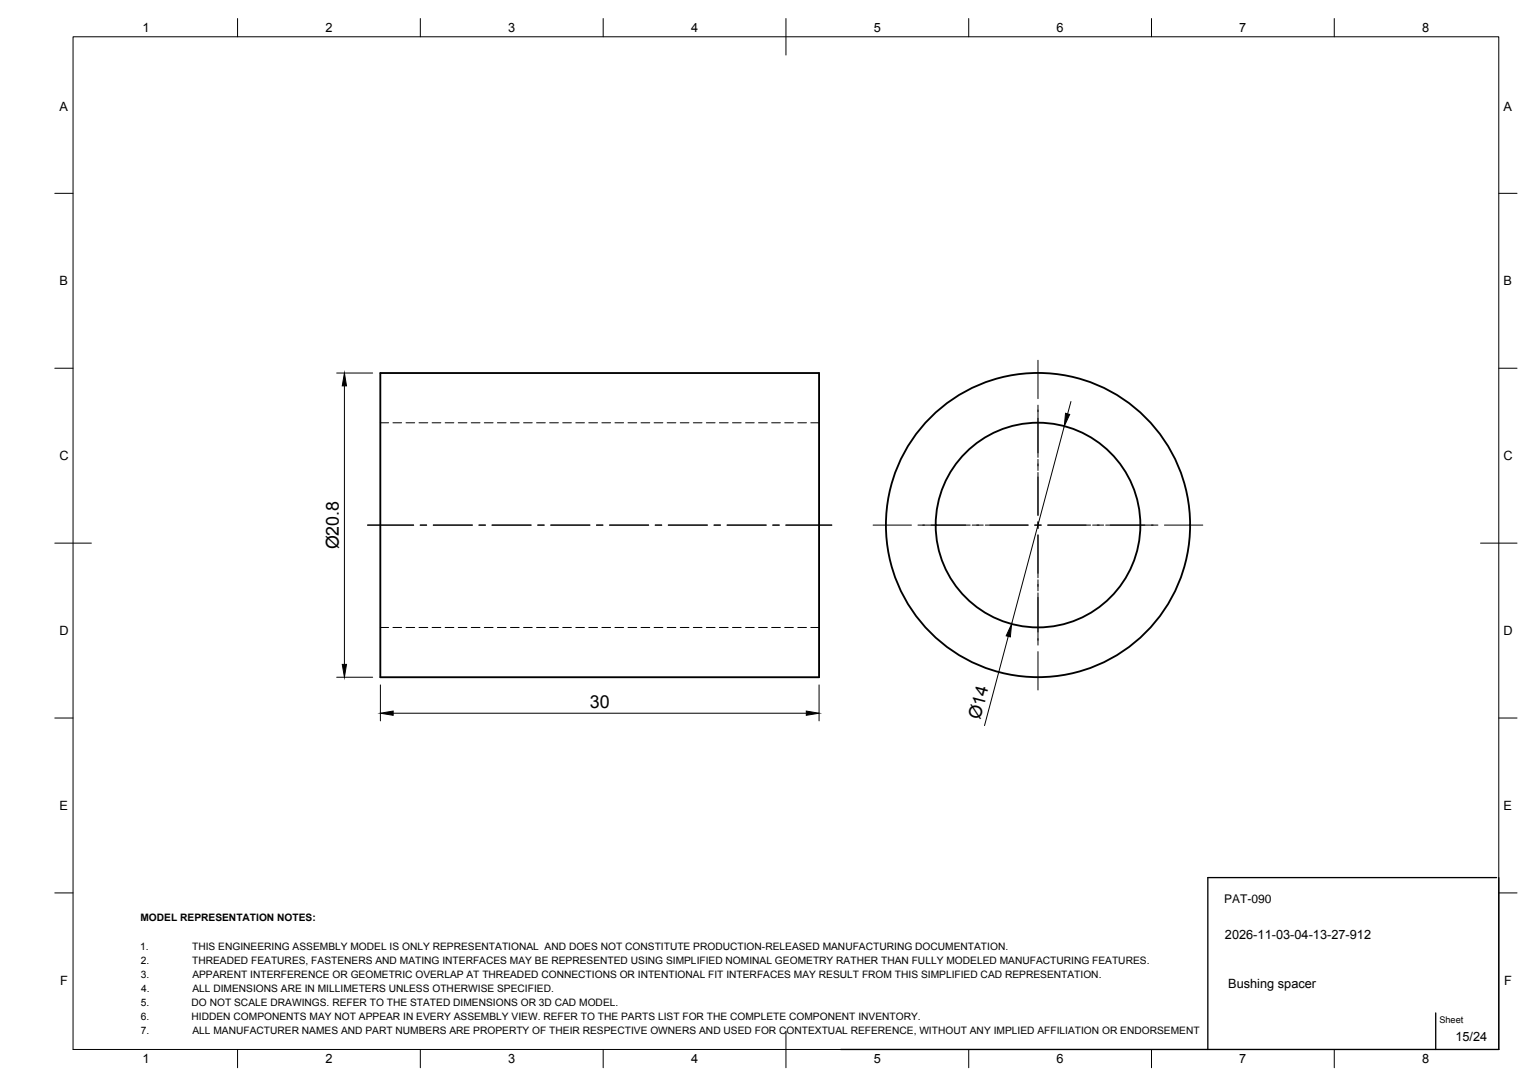
ISO-10303-21;
HEADER;
/* Generated by software containing ST-Developer
 * from STEP Tools, Inc. (www.steptools.com) 
 */

FILE_DESCRIPTION(
/* description */ ('Round-Shaft Linear Stage with Ball Bushings'),
/* implementation_level */ '2;1');

FILE_NAME(
/* name */ 'Bushing spacer.step',
/* time_stamp */ '2026-10-27T10:47:55-07:00',
/* author */ (''),
/* organization */ (''),
/* preprocessor_version */ 'ST-DEVELOPER v20.2',
/* originating_system */ 'Autodesk Translation Framework v15.17.0.0',
/* authorisation */ '');

FILE_SCHEMA (('AUTOMOTIVE_DESIGN { 1 0 10303 214 3 1 1 }'));
ENDSEC;

DATA;
#10=MECHANICAL_DESIGN_GEOMETRIC_PRESENTATION_REPRESENTATION('',(#311),#7835);
#269=SHAPE_REPRESENTATION_RELATIONSHIP('SRR','None',#7958,#290);
#290=ADVANCED_BREP_SHAPE_REPRESENTATION('',(#331),#7822);
#311=STYLED_ITEM('',(#8158),#331);
#331=MANIFOLD_SOLID_BREP('Body1',#4402);
#403=FACE_BOUND('',#1069,.T.);
#404=FACE_BOUND('',#1071,.T.);
#540=PLANE('',#4891);
#541=PLANE('',#4892);
#746=FACE_OUTER_BOUND('',#1066,.T.);
#747=FACE_OUTER_BOUND('',#1067,.T.);
#748=FACE_OUTER_BOUND('',#1068,.T.);
#749=FACE_OUTER_BOUND('',#1070,.T.);
#1066=EDGE_LOOP('',(#3542,#3543,#3544,#3545));
#1067=EDGE_LOOP('',(#3546,#3547,#3548,#3549));
#1068=EDGE_LOOP('',(#3550));
#1069=EDGE_LOOP('',(#3551));
#1070=EDGE_LOOP('',(#3552));
#1071=EDGE_LOOP('',(#3553));
#1430=LINE('',#7172,#1770);
#1431=LINE('',#7178,#1771);
#1770=VECTOR('',#5833,0.7);
#1771=VECTOR('',#5840,1.04);
#2022=CIRCLE('',#4886,0.7);
#2023=CIRCLE('',#4887,0.7);
#2024=CIRCLE('',#4889,1.04);
#2025=CIRCLE('',#4890,1.04);
#2299=VERTEX_POINT('',#7169);
#2300=VERTEX_POINT('',#7171);
#2301=VERTEX_POINT('',#7175);
#2302=VERTEX_POINT('',#7177);
#2739=EDGE_CURVE('',#2299,#2299,#2022,.T.);
#2740=EDGE_CURVE('',#2299,#2300,#1430,.T.);
#2741=EDGE_CURVE('',#2300,#2300,#2023,.T.);
#2742=EDGE_CURVE('',#2301,#2301,#2024,.T.);
#2743=EDGE_CURVE('',#2301,#2302,#1431,.T.);
#2744=EDGE_CURVE('',#2302,#2302,#2025,.T.);
#3542=ORIENTED_EDGE('',*,*,#2739,.F.);
#3543=ORIENTED_EDGE('',*,*,#2740,.T.);
#3544=ORIENTED_EDGE('',*,*,#2741,.T.);
#3545=ORIENTED_EDGE('',*,*,#2740,.F.);
#3546=ORIENTED_EDGE('',*,*,#2742,.F.);
#3547=ORIENTED_EDGE('',*,*,#2743,.T.);
#3548=ORIENTED_EDGE('',*,*,#2744,.T.);
#3549=ORIENTED_EDGE('',*,*,#2743,.F.);
#3550=ORIENTED_EDGE('',*,*,#2742,.T.);
#3551=ORIENTED_EDGE('',*,*,#2739,.T.);
#3552=ORIENTED_EDGE('',*,*,#2744,.F.);
#3553=ORIENTED_EDGE('',*,*,#2741,.F.);
#4096=CYLINDRICAL_SURFACE('',#4885,0.7);
#4097=CYLINDRICAL_SURFACE('',#4888,1.04);
#4265=ADVANCED_FACE('',(#746),#4096,.F.);
#4266=ADVANCED_FACE('',(#747),#4097,.T.);
#4267=ADVANCED_FACE('',(#748,#403),#540,.T.);
#4268=ADVANCED_FACE('',(#749,#404),#541,.F.);
#4402=CLOSED_SHELL('',(#4265,#4266,#4267,#4268));
#4884=AXIS2_PLACEMENT_3D('',#7167,#5827,#5828);
#4885=AXIS2_PLACEMENT_3D('',#7168,#5829,#5830);
#4886=AXIS2_PLACEMENT_3D('',#7170,#5831,#5832);
#4887=AXIS2_PLACEMENT_3D('',#7173,#5834,#5835);
#4888=AXIS2_PLACEMENT_3D('',#7174,#5836,#5837);
#4889=AXIS2_PLACEMENT_3D('',#7176,#5838,#5839);
#4890=AXIS2_PLACEMENT_3D('',#7179,#5841,#5842);
#4891=AXIS2_PLACEMENT_3D('',#7180,#5843,#5844);
#4892=AXIS2_PLACEMENT_3D('',#7181,#5845,#5846);
#5827=DIRECTION('axis',(0.,0.,1.));
#5828=DIRECTION('refdir',(1.,0.,0.));
#5829=DIRECTION('center_axis',(1.,0.,0.));
#5830=DIRECTION('ref_axis',(0.,0.,-1.));
#5831=DIRECTION('center_axis',(-1.,0.,0.));
#5832=DIRECTION('ref_axis',(0.,0.,-1.));
#5833=DIRECTION('',(-1.,0.,0.));
#5834=DIRECTION('center_axis',(-1.,0.,0.));
#5835=DIRECTION('ref_axis',(0.,0.,-1.));
#5836=DIRECTION('center_axis',(1.,0.,0.));
#5837=DIRECTION('ref_axis',(0.,0.,-1.));
#5838=DIRECTION('center_axis',(1.,0.,0.));
#5839=DIRECTION('ref_axis',(0.,0.,-1.));
#5840=DIRECTION('',(-1.,0.,0.));
#5841=DIRECTION('center_axis',(1.,0.,0.));
#5842=DIRECTION('ref_axis',(0.,0.,-1.));
#5843=DIRECTION('center_axis',(1.,0.,0.));
#5844=DIRECTION('ref_axis',(0.,0.,-1.));
#5845=DIRECTION('center_axis',(1.,0.,0.));
#5846=DIRECTION('ref_axis',(0.,0.,-1.));
#7167=CARTESIAN_POINT('',(0.,0.,0.));
#7168=CARTESIAN_POINT('Origin',(13.5,-4.,3.3));
#7169=CARTESIAN_POINT('',(16.5,-4.,4.));
#7170=CARTESIAN_POINT('Origin',(16.5,-4.,3.3));
#7171=CARTESIAN_POINT('',(13.5,-4.,4.));
#7172=CARTESIAN_POINT('',(13.5,-4.,4.));
#7173=CARTESIAN_POINT('Origin',(13.5,-4.,3.3));
#7174=CARTESIAN_POINT('Origin',(13.5,-4.,3.3));
#7175=CARTESIAN_POINT('',(16.5,-4.,4.34));
#7176=CARTESIAN_POINT('Origin',(16.5,-4.,3.3));
#7177=CARTESIAN_POINT('',(13.5,-4.,4.34));
#7178=CARTESIAN_POINT('',(13.5,-4.,4.34));
#7179=CARTESIAN_POINT('Origin',(13.5,-4.,3.3));
#7180=CARTESIAN_POINT('Origin',(16.5,-4.,3.3));
#7181=CARTESIAN_POINT('Origin',(13.5,-4.,3.3));
#7796=UNCERTAINTY_MEASURE_WITH_UNIT(LENGTH_MEASURE(0.001),#7836,
'DISTANCE_ACCURACY_VALUE',
'Maximum model space distance between geometric entities at asserted c
onnectivities');
#7809=UNCERTAINTY_MEASURE_WITH_UNIT(LENGTH_MEASURE(0.001),#7836,
'DISTANCE_ACCURACY_VALUE',
'Maximum model space distance between geometric entities at asserted c
onnectivities');
#7822=(
GEOMETRIC_REPRESENTATION_CONTEXT(3)
GLOBAL_UNCERTAINTY_ASSIGNED_CONTEXT((#7796))
GLOBAL_UNIT_ASSIGNED_CONTEXT((#7836,#7838,#7839))
REPRESENTATION_CONTEXT('','3D')
);
#7835=(
GEOMETRIC_REPRESENTATION_CONTEXT(3)
GLOBAL_UNCERTAINTY_ASSIGNED_CONTEXT((#7809))
GLOBAL_UNIT_ASSIGNED_CONTEXT((#7836,#7838,#7839))
REPRESENTATION_CONTEXT('','3D')
);
#7836=(
LENGTH_UNIT()
NAMED_UNIT(*)
SI_UNIT(.CENTI.,.METRE.)
);
#7838=(
NAMED_UNIT(*)
PLANE_ANGLE_UNIT()
SI_UNIT($,.RADIAN.)
);
#7839=(
NAMED_UNIT(*)
SI_UNIT($,.STERADIAN.)
SOLID_ANGLE_UNIT()
);
#7852=SHAPE_DEFINITION_REPRESENTATION(#7877,#7958);
#7877=PRODUCT_DEFINITION_SHAPE('',$,#7984);
#7958=SHAPE_REPRESENTATION('',(#4884),#7822);
#7971=PRODUCT_DEFINITION_CONTEXT('part definition',#8048,'design');
#7984=PRODUCT_DEFINITION('Bushing spacer','Bushing spacer',#8009,#7971);
#8009=PRODUCT_DEFINITION_FORMATION('',$,#8062);
#8048=APPLICATION_CONTEXT(
'Core Data for Automotive Mechanical Design Process');
#8049=PRODUCT_CONTEXT('part definition',#8048,'mechanical');
#8062=PRODUCT('Bushing spacer','Bushing spacer','Bushing spacer',(#8049));
#8152=COLOUR_RGB('Off White',0.89,0.88,0.83);
#8153=FILL_AREA_STYLE_COLOUR('',#8152);
#8154=FILL_AREA_STYLE('',(#8153));
#8155=SURFACE_STYLE_FILL_AREA(#8154);
#8156=SURFACE_SIDE_STYLE('',(#8155));
#8157=SURFACE_STYLE_USAGE(.BOTH.,#8156);
#8158=PRESENTATION_STYLE_ASSIGNMENT((#8157));
ENDSEC;
END-ISO-10303-21;
